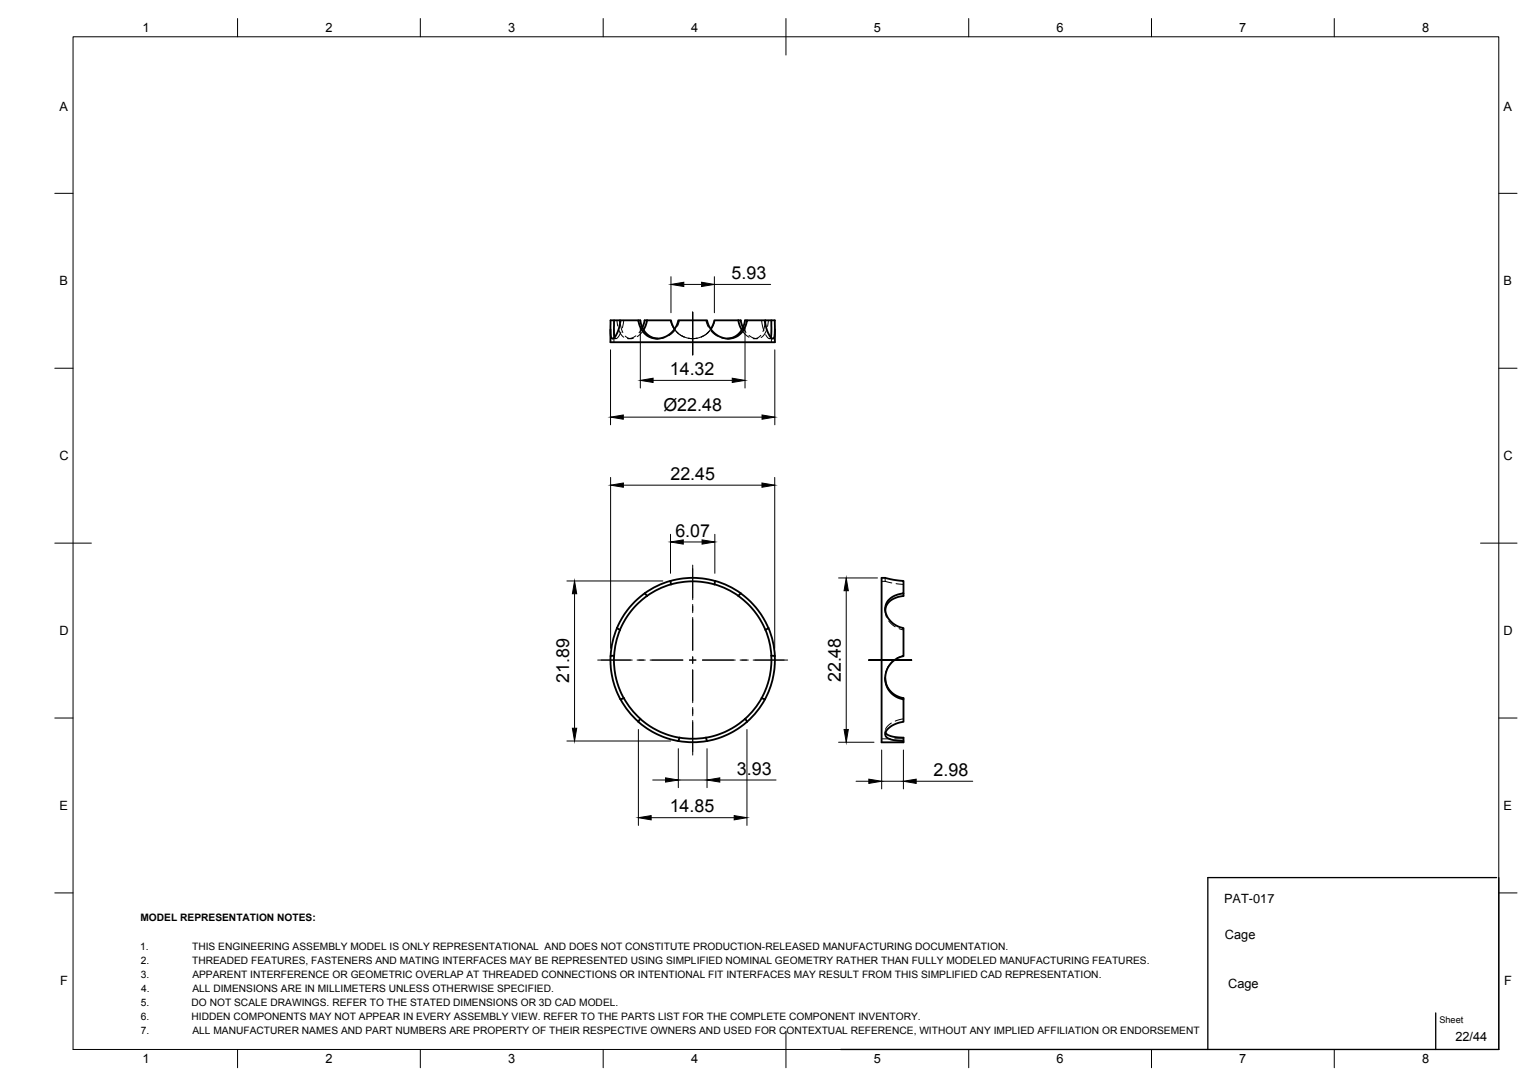
ISO-10303-21;
HEADER;
/* Generated by software containing ST-Developer
 * from STEP Tools, Inc. (www.steptools.com) 
 */

FILE_DESCRIPTION(
/* description */ ('Cam-and-follower valve demonstrator'),
/* implementation_level */ '2;1');

FILE_NAME(
/* name */ 'Cage.step',
/* time_stamp */ '2026-10-28T03:25:17-07:00',
/* author */ (''),
/* organization */ (''),
/* preprocessor_version */ 'ST-DEVELOPER v20.2',
/* originating_system */ 'Autodesk Translation Framework v15.17.0.0',
/* authorisation */ '');

FILE_SCHEMA (('AUTOMOTIVE_DESIGN { 1 0 10303 214 3 1 1 }'));
ENDSEC;

DATA;
#10=MECHANICAL_DESIGN_GEOMETRIC_PRESENTATION_REPRESENTATION('',(#433),#12896);
#300=SPHERICAL_SURFACE('',#6971,0.309556);
#301=SPHERICAL_SURFACE('',#6987,0.309556);
#302=SPHERICAL_SURFACE('',#6992,0.309556);
#303=SPHERICAL_SURFACE('',#6998,0.309556);
#304=SPHERICAL_SURFACE('',#7003,0.309556);
#305=SPHERICAL_SURFACE('',#7008,0.309556);
#306=SPHERICAL_SURFACE('',#7016,0.309556);
#325=B_SPLINE_CURVE_WITH_KNOTS('',3,(#11597,#11598,#11599,#11600,#11601,
#11602,#11603,#11604,#11605,#11606,#11607,#11608,#11609,#11610,#11611,#11612,
#11613,#11614,#11615,#11616,#11617,#11618),.UNSPECIFIED.,.F.,.F.,(4,2,2,
2,2,2,2,2,2,2,4),(0.0591825211272536,0.157966726598481,0.236950089897721,
0.315933453196962,0.391576304923761,0.46721915665056,0.54286200837736,0.618504860104159,
0.697488223403399,0.77647158670264,0.875255792173867),.UNSPECIFIED.);
#326=B_SPLINE_CURVE_WITH_KNOTS('',3,(#11622,#11623,#11624,#11625,#11626,
#11627,#11628,#11629,#11630,#11631,#11632,#11633,#11634,#11635,#11636,#11637,
#11638,#11639,#11640,#11641,#11642,#11643),.UNSPECIFIED.,.F.,.F.,(4,2,2,
2,2,2,2,2,2,2,4),(0.0581119756758434,0.106553146291161,0.213106292582322,
0.30849933801665,0.386091982889075,0.4636846277615,0.541277272633925,0.61886991750635,
0.714262962940678,0.820816109231839,0.869257279847157),.UNSPECIFIED.);
#327=B_SPLINE_CURVE_WITH_KNOTS('',3,(#11649,#11650,#11651,#11652,#11653,
#11654,#11655,#11656,#11657,#11658,#11659,#11660,#11661,#11662,#11663,#11664,
#11665,#11666,#11667,#11668,#11669,#11670),.UNSPECIFIED.,.F.,.F.,(4,2,2,
2,2,2,2,2,2,2,4),(0.0581119756758434,0.106553146291161,0.213106292582322,
0.30849933801665,0.386091982889075,0.4636846277615,0.541277272633925,0.61886991750635,
0.714262962940679,0.820816109231839,0.869257279847157),.UNSPECIFIED.);
#328=B_SPLINE_CURVE_WITH_KNOTS('',3,(#11674,#11675,#11676,#11677,#11678,
#11679,#11680,#11681,#11682,#11683,#11684,#11685,#11686,#11687,#11688,#11689,
#11690,#11691,#11692,#11693,#11694,#11695),.UNSPECIFIED.,.F.,.F.,(4,2,2,
2,2,2,2,2,2,2,4),(0.0581119756758433,0.106553146291161,0.213106292582322,
0.308499338016649,0.386091982889075,0.4636846277615,0.541277272633925,0.61886991750635,
0.714262962940678,0.820816109231839,0.869257279847157),.UNSPECIFIED.);
#329=B_SPLINE_CURVE_WITH_KNOTS('',3,(#11704,#11705,#11706,#11707,#11708,
#11709,#11710,#11711,#11712,#11713,#11714,#11715,#11716,#11717,#11718,#11719,
#11720,#11721,#11722,#11723,#11724,#11725),.UNSPECIFIED.,.F.,.F.,(4,2,2,
2,2,2,2,2,2,2,4),(0.0581119756758433,0.106553146291161,0.213106292582322,
0.30849933801665,0.386091982889075,0.4636846277615,0.541277272633925,0.61886991750635,
0.714262962940678,0.820816109231839,0.869257279847157),.UNSPECIFIED.);
#330=B_SPLINE_CURVE_WITH_KNOTS('',3,(#11729,#11730,#11731,#11732,#11733,
#11734,#11735,#11736,#11737,#11738,#11739,#11740,#11741,#11742,#11743,#11744,
#11745,#11746,#11747,#11748,#11749,#11750),.UNSPECIFIED.,.F.,.F.,(4,2,2,
2,2,2,2,2,2,2,4),(0.0581119756758434,0.106553146291161,0.213106292582322,
0.30849933801665,0.386091982889075,0.4636846277615,0.541277272633925,0.61886991750635,
0.714262962940678,0.820816109231839,0.869257279847157),.UNSPECIFIED.);
#331=B_SPLINE_CURVE_WITH_KNOTS('',3,(#11754,#11755,#11756,#11757,#11758,
#11759,#11760,#11761,#11762,#11763,#11764,#11765,#11766,#11767,#11768,#11769,
#11770,#11771,#11772,#11773,#11774,#11775),.UNSPECIFIED.,.F.,.F.,(4,2,2,
2,2,2,2,2,2,2,4),(0.0581119756758434,0.106553146291161,0.213106292582322,
0.30849933801665,0.386091982889075,0.4636846277615,0.541277272633925,0.61886991750635,
0.714262962940678,0.820816109231839,0.869257279847157),.UNSPECIFIED.);
#332=B_SPLINE_CURVE_WITH_KNOTS('',3,(#11779,#11780,#11781,#11782,#11783,
#11784,#11785,#11786,#11787,#11788,#11789,#11790,#11791,#11792,#11793,#11794,
#11795,#11796,#11797,#11798,#11799,#11800),.UNSPECIFIED.,.F.,.F.,(4,2,2,
2,2,2,2,2,2,2,4),(0.0581119756758433,0.106553146291161,0.213106292582322,
0.30849933801665,0.386091982889075,0.4636846277615,0.541277272633925,0.61886991750635,
0.714262962940678,0.820816109231839,0.869257279847157),.UNSPECIFIED.);
#333=B_SPLINE_CURVE_WITH_KNOTS('',3,(#11808,#11809,#11810,#11811,#11812,
#11813,#11814,#11815,#11816,#11817,#11818,#11819,#11820,#11821,#11822,#11823,
#11824,#11825,#11826,#11827,#11828,#11829),.UNSPECIFIED.,.F.,.F.,(4,2,2,
2,2,2,2,2,2,2,4),(0.0591825211272536,0.157966726598481,0.236950089897721,
0.315933453196962,0.391576304923761,0.467219156650561,0.54286200837736,
0.618504860104159,0.697488223403399,0.77647158670264,0.875255792173867),
 .UNSPECIFIED.);
#334=B_SPLINE_CURVE_WITH_KNOTS('',3,(#11837,#11838,#11839,#11840,#11841,
#11842,#11843,#11844,#11845,#11846,#11847,#11848,#11849,#11850,#11851,#11852,
#11853,#11854,#11855,#11856,#11857,#11858),.UNSPECIFIED.,.F.,.F.,(4,2,2,
2,2,2,2,2,2,2,4),(0.0591825211272536,0.157966726598481,0.236950089897722,
0.315933453196962,0.391576304923761,0.467219156650561,0.54286200837736,
0.618504860104159,0.697488223403399,0.77647158670264,0.875255792173867),
 .UNSPECIFIED.);
#335=B_SPLINE_CURVE_WITH_KNOTS('',3,(#11868,#11869,#11870,#11871,#11872,
#11873,#11874,#11875,#11876,#11877,#11878,#11879,#11880,#11881,#11882,#11883,
#11884,#11885,#11886,#11887,#11888,#11889),.UNSPECIFIED.,.F.,.F.,(4,2,2,
2,2,2,2,2,2,2,4),(0.0591825211272536,0.157966726598481,0.236950089897721,
0.315933453196962,0.391576304923761,0.46721915665056,0.54286200837736,0.618504860104159,
0.697488223403399,0.77647158670264,0.875255792173867),.UNSPECIFIED.);
#336=B_SPLINE_CURVE_WITH_KNOTS('',3,(#11897,#11898,#11899,#11900,#11901,
#11902,#11903,#11904,#11905,#11906,#11907,#11908,#11909,#11910,#11911,#11912,
#11913,#11914,#11915,#11916,#11917,#11918),.UNSPECIFIED.,.F.,.F.,(4,2,2,
2,2,2,2,2,2,2,4),(0.0591825211272536,0.157966726598481,0.236950089897721,
0.315933453196962,0.391576304923761,0.46721915665056,0.542862008377359,
0.618504860104159,0.697488223403399,0.776471586702639,0.875255792173867),
 .UNSPECIFIED.);
#337=B_SPLINE_CURVE_WITH_KNOTS('',3,(#11926,#11927,#11928,#11929,#11930,
#11931,#11932,#11933,#11934,#11935,#11936,#11937,#11938,#11939,#11940,#11941,
#11942,#11943,#11944,#11945,#11946,#11947),.UNSPECIFIED.,.F.,.F.,(4,2,2,
2,2,2,2,2,2,2,4),(0.0591825211272536,0.157966726598481,0.236950089897721,
0.315933453196962,0.391576304923761,0.46721915665056,0.54286200837736,0.618504860104159,
0.697488223403399,0.77647158670264,0.875255792173867),.UNSPECIFIED.);
#338=B_SPLINE_CURVE_WITH_KNOTS('',3,(#11956,#11957,#11958,#11959,#11960,
#11961,#11962,#11963,#11964,#11965,#11966,#11967,#11968,#11969,#11970,#11971,
#11972,#11973,#11974,#11975,#11976,#11977),.UNSPECIFIED.,.F.,.F.,(4,2,2,
2,2,2,2,2,2,2,4),(0.0591825211272536,0.157966726598481,0.236950089897721,
0.315933453196962,0.391576304923761,0.46721915665056,0.542862008377359,
0.618504860104159,0.697488223403399,0.776471586702639,0.875255792173867),
 .UNSPECIFIED.);
#355=SHAPE_REPRESENTATION_RELATIONSHIP('SRR','None',#13072,#391);
#391=ADVANCED_BREP_SHAPE_REPRESENTATION('',(#476),#12872);
#433=STYLED_ITEM('',(#13330),#476);
#476=MANIFOLD_SOLID_BREP('Continuous crown cage',#6200);
#608=FACE_BOUND('',#1762,.T.);
#820=CIRCLE('',#6972,0.303778037777585);
#821=CIRCLE('',#6973,0.303778037777585);
#822=CIRCLE('',#6975,1.123812);
#823=CIRCLE('',#6976,1.123812);
#824=CIRCLE('',#6977,1.123812);
#825=CIRCLE('',#6978,1.123812);
#826=CIRCLE('',#6979,1.123812);
#827=CIRCLE('',#6980,1.123812);
#828=CIRCLE('',#6981,1.123812);
#829=CIRCLE('',#6982,1.123812);
#830=CIRCLE('',#6983,1.123812);
#831=CIRCLE('',#6985,1.076188);
#832=CIRCLE('',#6986,0.303778037777585);
#833=CIRCLE('',#6988,0.303778037777585);
#834=CIRCLE('',#6990,1.076188);
#835=CIRCLE('',#6991,0.303778037777585);
#836=CIRCLE('',#6993,0.303778037777585);
#837=CIRCLE('',#6995,1.076188);
#838=CIRCLE('',#6996,1.076188);
#839=CIRCLE('',#6997,0.303778037777585);
#840=CIRCLE('',#6999,0.303778037777585);
#841=CIRCLE('',#7001,1.076188);
#842=CIRCLE('',#7002,0.303778037777585);
#843=CIRCLE('',#7004,0.303778037777585);
#844=CIRCLE('',#7006,1.076188);
#845=CIRCLE('',#7007,0.303778037777585);
#846=CIRCLE('',#7009,0.303778037777585);
#847=CIRCLE('',#7011,1.076188);
#848=CIRCLE('',#7012,1.076188);
#849=CIRCLE('',#7013,1.076188);
#850=CIRCLE('',#7015,0.303778037777585);
#851=CIRCLE('',#7017,0.303778037777585);
#1044=CYLINDRICAL_SURFACE('',#6974,1.123812);
#1045=CYLINDRICAL_SURFACE('',#7010,1.076188);
#1265=FACE_OUTER_BOUND('',#1746,.T.);
#1266=FACE_OUTER_BOUND('',#1747,.T.);
#1267=FACE_OUTER_BOUND('',#1748,.T.);
#1268=FACE_OUTER_BOUND('',#1749,.T.);
#1269=FACE_OUTER_BOUND('',#1750,.T.);
#1270=FACE_OUTER_BOUND('',#1751,.T.);
#1271=FACE_OUTER_BOUND('',#1752,.T.);
#1272=FACE_OUTER_BOUND('',#1753,.T.);
#1273=FACE_OUTER_BOUND('',#1754,.T.);
#1274=FACE_OUTER_BOUND('',#1755,.T.);
#1275=FACE_OUTER_BOUND('',#1756,.T.);
#1276=FACE_OUTER_BOUND('',#1757,.T.);
#1277=FACE_OUTER_BOUND('',#1758,.T.);
#1278=FACE_OUTER_BOUND('',#1759,.T.);
#1279=FACE_OUTER_BOUND('',#1760,.T.);
#1280=FACE_OUTER_BOUND('',#1761,.T.);
#1281=FACE_OUTER_BOUND('',#1763,.T.);
#1746=EDGE_LOOP('',(#4833,#4834,#4835,#4836));
#1747=EDGE_LOOP('',(#4837,#4838,#4839,#4840,#4841,#4842,#4843,#4844,#4845,
#4846,#4847,#4848,#4849,#4850,#4851,#4852,#4853,#4854));
#1748=EDGE_LOOP('',(#4855,#4856,#4857,#4858));
#1749=EDGE_LOOP('',(#4859,#4860,#4861,#4862));
#1750=EDGE_LOOP('',(#4863,#4864,#4865,#4866));
#1751=EDGE_LOOP('',(#4867,#4868,#4869,#4870));
#1752=EDGE_LOOP('',(#4871,#4872,#4873,#4874,#4875,#4876));
#1753=EDGE_LOOP('',(#4877,#4878,#4879,#4880));
#1754=EDGE_LOOP('',(#4881,#4882,#4883,#4884));
#1755=EDGE_LOOP('',(#4885,#4886,#4887,#4888));
#1756=EDGE_LOOP('',(#4889,#4890,#4891,#4892));
#1757=EDGE_LOOP('',(#4893,#4894,#4895,#4896));
#1758=EDGE_LOOP('',(#4897,#4898,#4899,#4900,#4901,#4902,#4903,#4904,#4905,
#4906,#4907,#4908,#4909,#4910,#4911,#4912,#4913,#4914));
#1759=EDGE_LOOP('',(#4915,#4916,#4917,#4918));
#1760=EDGE_LOOP('',(#4919,#4920,#4921,#4922));
#1761=EDGE_LOOP('',(#4923));
#1762=EDGE_LOOP('',(#4924));
#1763=EDGE_LOOP('',(#4925,#4926,#4927,#4928));
#2202=LINE('',#11699,#2624);
#2203=LINE('',#11952,#2625);
#2624=VECTOR('',#8333,1.123812);
#2625=VECTOR('',#8402,1.076188);
#3093=VERTEX_POINT('',#11595);
#3094=VERTEX_POINT('',#11596);
#3095=VERTEX_POINT('',#11619);
#3096=VERTEX_POINT('',#11621);
#3097=VERTEX_POINT('',#11646);
#3098=VERTEX_POINT('',#11648);
#3099=VERTEX_POINT('',#11671);
#3100=VERTEX_POINT('',#11673);
#3101=VERTEX_POINT('',#11696);
#3102=VERTEX_POINT('',#11698);
#3103=VERTEX_POINT('',#11701);
#3104=VERTEX_POINT('',#11703);
#3105=VERTEX_POINT('',#11726);
#3106=VERTEX_POINT('',#11728);
#3107=VERTEX_POINT('',#11751);
#3108=VERTEX_POINT('',#11753);
#3109=VERTEX_POINT('',#11776);
#3110=VERTEX_POINT('',#11778);
#3111=VERTEX_POINT('',#11803);
#3112=VERTEX_POINT('',#11807);
#3113=VERTEX_POINT('',#11832);
#3114=VERTEX_POINT('',#11836);
#3115=VERTEX_POINT('',#11861);
#3116=VERTEX_POINT('',#11863);
#3117=VERTEX_POINT('',#11867);
#3118=VERTEX_POINT('',#11892);
#3119=VERTEX_POINT('',#11896);
#3120=VERTEX_POINT('',#11921);
#3121=VERTEX_POINT('',#11925);
#3122=VERTEX_POINT('',#11950);
#3123=VERTEX_POINT('',#11953);
#3124=VERTEX_POINT('',#11955);
#3713=EDGE_CURVE('',#3093,#3094,#325,.T.);
#3714=EDGE_CURVE('',#3095,#3093,#820,.T.);
#3715=EDGE_CURVE('',#3096,#3095,#326,.T.);
#3716=EDGE_CURVE('',#3094,#3096,#821,.T.);
#3717=EDGE_CURVE('',#3097,#3095,#822,.T.);
#3718=EDGE_CURVE('',#3097,#3098,#327,.T.);
#3719=EDGE_CURVE('',#3099,#3098,#823,.T.);
#3720=EDGE_CURVE('',#3099,#3100,#328,.T.);
#3721=EDGE_CURVE('',#3101,#3100,#824,.T.);
#3722=EDGE_CURVE('',#3101,#3102,#2202,.T.);
#3723=EDGE_CURVE('',#3102,#3102,#825,.T.);
#3724=EDGE_CURVE('',#3103,#3101,#826,.T.);
#3725=EDGE_CURVE('',#3103,#3104,#329,.T.);
#3726=EDGE_CURVE('',#3105,#3104,#827,.T.);
#3727=EDGE_CURVE('',#3105,#3106,#330,.T.);
#3728=EDGE_CURVE('',#3107,#3106,#828,.T.);
#3729=EDGE_CURVE('',#3107,#3108,#331,.T.);
#3730=EDGE_CURVE('',#3109,#3108,#829,.T.);
#3731=EDGE_CURVE('',#3109,#3110,#332,.T.);
#3732=EDGE_CURVE('',#3096,#3110,#830,.T.);
#3733=EDGE_CURVE('',#3093,#3111,#831,.T.);
#3734=EDGE_CURVE('',#3111,#3097,#832,.T.);
#3735=EDGE_CURVE('',#3112,#3111,#333,.T.);
#3736=EDGE_CURVE('',#3098,#3112,#833,.T.);
#3737=EDGE_CURVE('',#3112,#3113,#834,.T.);
#3738=EDGE_CURVE('',#3113,#3099,#835,.T.);
#3739=EDGE_CURVE('',#3114,#3113,#334,.T.);
#3740=EDGE_CURVE('',#3100,#3114,#836,.T.);
#3741=EDGE_CURVE('',#3114,#3115,#837,.T.);
#3742=EDGE_CURVE('',#3115,#3116,#838,.T.);
#3743=EDGE_CURVE('',#3116,#3103,#839,.T.);
#3744=EDGE_CURVE('',#3117,#3116,#335,.T.);
#3745=EDGE_CURVE('',#3104,#3117,#840,.T.);
#3746=EDGE_CURVE('',#3117,#3118,#841,.T.);
#3747=EDGE_CURVE('',#3118,#3105,#842,.T.);
#3748=EDGE_CURVE('',#3119,#3118,#336,.T.);
#3749=EDGE_CURVE('',#3106,#3119,#843,.T.);
#3750=EDGE_CURVE('',#3119,#3120,#844,.T.);
#3751=EDGE_CURVE('',#3120,#3107,#845,.T.);
#3752=EDGE_CURVE('',#3121,#3120,#337,.T.);
#3753=EDGE_CURVE('',#3108,#3121,#846,.T.);
#3754=EDGE_CURVE('',#3122,#3122,#847,.T.);
#3755=EDGE_CURVE('',#3122,#3115,#2203,.T.);
#3756=EDGE_CURVE('',#3123,#3094,#848,.T.);
#3757=EDGE_CURVE('',#3123,#3124,#338,.T.);
#3758=EDGE_CURVE('',#3121,#3124,#849,.T.);
#3759=EDGE_CURVE('',#3110,#3123,#850,.T.);
#3760=EDGE_CURVE('',#3124,#3109,#851,.T.);
#4833=ORIENTED_EDGE('',*,*,#3713,.F.);
#4834=ORIENTED_EDGE('',*,*,#3714,.F.);
#4835=ORIENTED_EDGE('',*,*,#3715,.F.);
#4836=ORIENTED_EDGE('',*,*,#3716,.F.);
#4837=ORIENTED_EDGE('',*,*,#3715,.T.);
#4838=ORIENTED_EDGE('',*,*,#3717,.F.);
#4839=ORIENTED_EDGE('',*,*,#3718,.T.);
#4840=ORIENTED_EDGE('',*,*,#3719,.F.);
#4841=ORIENTED_EDGE('',*,*,#3720,.T.);
#4842=ORIENTED_EDGE('',*,*,#3721,.F.);
#4843=ORIENTED_EDGE('',*,*,#3722,.T.);
#4844=ORIENTED_EDGE('',*,*,#3723,.F.);
#4845=ORIENTED_EDGE('',*,*,#3722,.F.);
#4846=ORIENTED_EDGE('',*,*,#3724,.F.);
#4847=ORIENTED_EDGE('',*,*,#3725,.T.);
#4848=ORIENTED_EDGE('',*,*,#3726,.F.);
#4849=ORIENTED_EDGE('',*,*,#3727,.T.);
#4850=ORIENTED_EDGE('',*,*,#3728,.F.);
#4851=ORIENTED_EDGE('',*,*,#3729,.T.);
#4852=ORIENTED_EDGE('',*,*,#3730,.F.);
#4853=ORIENTED_EDGE('',*,*,#3731,.T.);
#4854=ORIENTED_EDGE('',*,*,#3732,.F.);
#4855=ORIENTED_EDGE('',*,*,#3714,.T.);
#4856=ORIENTED_EDGE('',*,*,#3733,.T.);
#4857=ORIENTED_EDGE('',*,*,#3734,.T.);
#4858=ORIENTED_EDGE('',*,*,#3717,.T.);
#4859=ORIENTED_EDGE('',*,*,#3735,.F.);
#4860=ORIENTED_EDGE('',*,*,#3736,.F.);
#4861=ORIENTED_EDGE('',*,*,#3718,.F.);
#4862=ORIENTED_EDGE('',*,*,#3734,.F.);
#4863=ORIENTED_EDGE('',*,*,#3736,.T.);
#4864=ORIENTED_EDGE('',*,*,#3737,.T.);
#4865=ORIENTED_EDGE('',*,*,#3738,.T.);
#4866=ORIENTED_EDGE('',*,*,#3719,.T.);
#4867=ORIENTED_EDGE('',*,*,#3739,.F.);
#4868=ORIENTED_EDGE('',*,*,#3740,.F.);
#4869=ORIENTED_EDGE('',*,*,#3720,.F.);
#4870=ORIENTED_EDGE('',*,*,#3738,.F.);
#4871=ORIENTED_EDGE('',*,*,#3740,.T.);
#4872=ORIENTED_EDGE('',*,*,#3741,.T.);
#4873=ORIENTED_EDGE('',*,*,#3742,.T.);
#4874=ORIENTED_EDGE('',*,*,#3743,.T.);
#4875=ORIENTED_EDGE('',*,*,#3724,.T.);
#4876=ORIENTED_EDGE('',*,*,#3721,.T.);
#4877=ORIENTED_EDGE('',*,*,#3744,.F.);
#4878=ORIENTED_EDGE('',*,*,#3745,.F.);
#4879=ORIENTED_EDGE('',*,*,#3725,.F.);
#4880=ORIENTED_EDGE('',*,*,#3743,.F.);
#4881=ORIENTED_EDGE('',*,*,#3745,.T.);
#4882=ORIENTED_EDGE('',*,*,#3746,.T.);
#4883=ORIENTED_EDGE('',*,*,#3747,.T.);
#4884=ORIENTED_EDGE('',*,*,#3726,.T.);
#4885=ORIENTED_EDGE('',*,*,#3748,.F.);
#4886=ORIENTED_EDGE('',*,*,#3749,.F.);
#4887=ORIENTED_EDGE('',*,*,#3727,.F.);
#4888=ORIENTED_EDGE('',*,*,#3747,.F.);
#4889=ORIENTED_EDGE('',*,*,#3749,.T.);
#4890=ORIENTED_EDGE('',*,*,#3750,.T.);
#4891=ORIENTED_EDGE('',*,*,#3751,.T.);
#4892=ORIENTED_EDGE('',*,*,#3728,.T.);
#4893=ORIENTED_EDGE('',*,*,#3729,.F.);
#4894=ORIENTED_EDGE('',*,*,#3751,.F.);
#4895=ORIENTED_EDGE('',*,*,#3752,.F.);
#4896=ORIENTED_EDGE('',*,*,#3753,.F.);
#4897=ORIENTED_EDGE('',*,*,#3754,.F.);
#4898=ORIENTED_EDGE('',*,*,#3755,.T.);
#4899=ORIENTED_EDGE('',*,*,#3741,.F.);
#4900=ORIENTED_EDGE('',*,*,#3739,.T.);
#4901=ORIENTED_EDGE('',*,*,#3737,.F.);
#4902=ORIENTED_EDGE('',*,*,#3735,.T.);
#4903=ORIENTED_EDGE('',*,*,#3733,.F.);
#4904=ORIENTED_EDGE('',*,*,#3713,.T.);
#4905=ORIENTED_EDGE('',*,*,#3756,.F.);
#4906=ORIENTED_EDGE('',*,*,#3757,.T.);
#4907=ORIENTED_EDGE('',*,*,#3758,.F.);
#4908=ORIENTED_EDGE('',*,*,#3752,.T.);
#4909=ORIENTED_EDGE('',*,*,#3750,.F.);
#4910=ORIENTED_EDGE('',*,*,#3748,.T.);
#4911=ORIENTED_EDGE('',*,*,#3746,.F.);
#4912=ORIENTED_EDGE('',*,*,#3744,.T.);
#4913=ORIENTED_EDGE('',*,*,#3742,.F.);
#4914=ORIENTED_EDGE('',*,*,#3755,.F.);
#4915=ORIENTED_EDGE('',*,*,#3716,.T.);
#4916=ORIENTED_EDGE('',*,*,#3732,.T.);
#4917=ORIENTED_EDGE('',*,*,#3759,.T.);
#4918=ORIENTED_EDGE('',*,*,#3756,.T.);
#4919=ORIENTED_EDGE('',*,*,#3731,.F.);
#4920=ORIENTED_EDGE('',*,*,#3760,.F.);
#4921=ORIENTED_EDGE('',*,*,#3757,.F.);
#4922=ORIENTED_EDGE('',*,*,#3759,.F.);
#4923=ORIENTED_EDGE('',*,*,#3723,.T.);
#4924=ORIENTED_EDGE('',*,*,#3754,.T.);
#4925=ORIENTED_EDGE('',*,*,#3753,.T.);
#4926=ORIENTED_EDGE('',*,*,#3758,.T.);
#4927=ORIENTED_EDGE('',*,*,#3760,.T.);
#4928=ORIENTED_EDGE('',*,*,#3730,.T.);
#5682=PLANE('',#6984);
#5683=PLANE('',#6989);
#5684=PLANE('',#6994);
#5685=PLANE('',#7000);
#5686=PLANE('',#7005);
#5687=PLANE('',#7014);
#5688=PLANE('',#7018);
#5689=PLANE('',#7019);
#5981=ADVANCED_FACE('',(#1265),#300,.F.);
#5982=ADVANCED_FACE('',(#1266),#1044,.T.);
#5983=ADVANCED_FACE('',(#1267),#5682,.T.);
#5984=ADVANCED_FACE('',(#1268),#301,.F.);
#5985=ADVANCED_FACE('',(#1269),#5683,.T.);
#5986=ADVANCED_FACE('',(#1270),#302,.F.);
#5987=ADVANCED_FACE('',(#1271),#5684,.T.);
#5988=ADVANCED_FACE('',(#1272),#303,.F.);
#5989=ADVANCED_FACE('',(#1273),#5685,.T.);
#5990=ADVANCED_FACE('',(#1274),#304,.F.);
#5991=ADVANCED_FACE('',(#1275),#5686,.T.);
#5992=ADVANCED_FACE('',(#1276),#305,.F.);
#5993=ADVANCED_FACE('',(#1277),#1045,.F.);
#5994=ADVANCED_FACE('',(#1278),#5687,.T.);
#5995=ADVANCED_FACE('',(#1279),#306,.F.);
#5996=ADVANCED_FACE('',(#1280,#608),#5688,.T.);
#5997=ADVANCED_FACE('',(#1281),#5689,.T.);
#6200=CLOSED_SHELL('',(#5981,#5982,#5983,#5984,#5985,#5986,#5987,#5988,
#5989,#5990,#5991,#5992,#5993,#5994,#5995,#5996,#5997));
#6970=AXIS2_PLACEMENT_3D('',#11593,#8317,#8318);
#6971=AXIS2_PLACEMENT_3D('',#11594,#8319,#8320);
#6972=AXIS2_PLACEMENT_3D('',#11620,#8321,#8322);
#6973=AXIS2_PLACEMENT_3D('',#11644,#8323,#8324);
#6974=AXIS2_PLACEMENT_3D('',#11645,#8325,#8326);
#6975=AXIS2_PLACEMENT_3D('',#11647,#8327,#8328);
#6976=AXIS2_PLACEMENT_3D('',#11672,#8329,#8330);
#6977=AXIS2_PLACEMENT_3D('',#11697,#8331,#8332);
#6978=AXIS2_PLACEMENT_3D('',#11700,#8334,#8335);
#6979=AXIS2_PLACEMENT_3D('',#11702,#8336,#8337);
#6980=AXIS2_PLACEMENT_3D('',#11727,#8338,#8339);
#6981=AXIS2_PLACEMENT_3D('',#11752,#8340,#8341);
#6982=AXIS2_PLACEMENT_3D('',#11777,#8342,#8343);
#6983=AXIS2_PLACEMENT_3D('',#11801,#8344,#8345);
#6984=AXIS2_PLACEMENT_3D('',#11802,#8346,#8347);
#6985=AXIS2_PLACEMENT_3D('',#11804,#8348,#8349);
#6986=AXIS2_PLACEMENT_3D('',#11805,#8350,#8351);
#6987=AXIS2_PLACEMENT_3D('',#11806,#8352,#8353);
#6988=AXIS2_PLACEMENT_3D('',#11830,#8354,#8355);
#6989=AXIS2_PLACEMENT_3D('',#11831,#8356,#8357);
#6990=AXIS2_PLACEMENT_3D('',#11833,#8358,#8359);
#6991=AXIS2_PLACEMENT_3D('',#11834,#8360,#8361);
#6992=AXIS2_PLACEMENT_3D('',#11835,#8362,#8363);
#6993=AXIS2_PLACEMENT_3D('',#11859,#8364,#8365);
#6994=AXIS2_PLACEMENT_3D('',#11860,#8366,#8367);
#6995=AXIS2_PLACEMENT_3D('',#11862,#8368,#8369);
#6996=AXIS2_PLACEMENT_3D('',#11864,#8370,#8371);
#6997=AXIS2_PLACEMENT_3D('',#11865,#8372,#8373);
#6998=AXIS2_PLACEMENT_3D('',#11866,#8374,#8375);
#6999=AXIS2_PLACEMENT_3D('',#11890,#8376,#8377);
#7000=AXIS2_PLACEMENT_3D('',#11891,#8378,#8379);
#7001=AXIS2_PLACEMENT_3D('',#11893,#8380,#8381);
#7002=AXIS2_PLACEMENT_3D('',#11894,#8382,#8383);
#7003=AXIS2_PLACEMENT_3D('',#11895,#8384,#8385);
#7004=AXIS2_PLACEMENT_3D('',#11919,#8386,#8387);
#7005=AXIS2_PLACEMENT_3D('',#11920,#8388,#8389);
#7006=AXIS2_PLACEMENT_3D('',#11922,#8390,#8391);
#7007=AXIS2_PLACEMENT_3D('',#11923,#8392,#8393);
#7008=AXIS2_PLACEMENT_3D('',#11924,#8394,#8395);
#7009=AXIS2_PLACEMENT_3D('',#11948,#8396,#8397);
#7010=AXIS2_PLACEMENT_3D('',#11949,#8398,#8399);
#7011=AXIS2_PLACEMENT_3D('',#11951,#8400,#8401);
#7012=AXIS2_PLACEMENT_3D('',#11954,#8403,#8404);
#7013=AXIS2_PLACEMENT_3D('',#11978,#8405,#8406);
#7014=AXIS2_PLACEMENT_3D('',#11979,#8407,#8408);
#7015=AXIS2_PLACEMENT_3D('',#11980,#8409,#8410);
#7016=AXIS2_PLACEMENT_3D('',#11981,#8411,#8412);
#7017=AXIS2_PLACEMENT_3D('',#11982,#8413,#8414);
#7018=AXIS2_PLACEMENT_3D('',#11983,#8415,#8416);
#7019=AXIS2_PLACEMENT_3D('',#11984,#8417,#8418);
#8317=DIRECTION('axis',(0.,0.,1.));
#8318=DIRECTION('refdir',(1.,0.,0.));
#8319=DIRECTION('center_axis',(0.,0.,1.));
#8320=DIRECTION('ref_axis',(1.,0.,0.));
#8321=DIRECTION('center_axis',(0.,-1.,0.));
#8322=DIRECTION('ref_axis',(0.,0.,-1.));
#8323=DIRECTION('center_axis',(0.,-1.,0.));
#8324=DIRECTION('ref_axis',(0.,0.,-1.));
#8325=DIRECTION('center_axis',(0.,1.,0.));
#8326=DIRECTION('ref_axis',(1.,0.,0.));
#8327=DIRECTION('center_axis',(0.,1.,0.));
#8328=DIRECTION('ref_axis',(1.,0.,0.));
#8329=DIRECTION('center_axis',(0.,1.,0.));
#8330=DIRECTION('ref_axis',(1.,0.,0.));
#8331=DIRECTION('center_axis',(0.,1.,0.));
#8332=DIRECTION('ref_axis',(1.,0.,0.));
#8333=DIRECTION('',(0.,-1.,0.));
#8334=DIRECTION('center_axis',(0.,-1.,0.));
#8335=DIRECTION('ref_axis',(1.,0.,0.));
#8336=DIRECTION('center_axis',(0.,1.,0.));
#8337=DIRECTION('ref_axis',(1.,0.,0.));
#8338=DIRECTION('center_axis',(0.,1.,0.));
#8339=DIRECTION('ref_axis',(1.,0.,0.));
#8340=DIRECTION('center_axis',(0.,1.,0.));
#8341=DIRECTION('ref_axis',(1.,0.,0.));
#8342=DIRECTION('center_axis',(0.,1.,0.));
#8343=DIRECTION('ref_axis',(1.,0.,0.));
#8344=DIRECTION('center_axis',(0.,1.,0.));
#8345=DIRECTION('ref_axis',(1.,0.,0.));
#8346=DIRECTION('center_axis',(0.,1.,0.));
#8347=DIRECTION('ref_axis',(1.,0.,0.));
#8348=DIRECTION('center_axis',(0.,-1.,0.));
#8349=DIRECTION('ref_axis',(1.,0.,0.));
#8350=DIRECTION('center_axis',(0.,-1.,0.));
#8351=DIRECTION('ref_axis',(0.,0.,-1.));
#8352=DIRECTION('center_axis',(8.96625347776458E-17,0.,1.));
#8353=DIRECTION('ref_axis',(1.,0.,0.));
#8354=DIRECTION('center_axis',(0.,-1.,0.));
#8355=DIRECTION('ref_axis',(0.,0.,-1.));
#8356=DIRECTION('center_axis',(0.,1.,0.));
#8357=DIRECTION('ref_axis',(1.,0.,0.));
#8358=DIRECTION('center_axis',(0.,-1.,0.));
#8359=DIRECTION('ref_axis',(1.,0.,0.));
#8360=DIRECTION('center_axis',(0.,-1.,0.));
#8361=DIRECTION('ref_axis',(0.,0.,-1.));
#8362=DIRECTION('center_axis',(0.,0.,1.));
#8363=DIRECTION('ref_axis',(1.,0.,0.));
#8364=DIRECTION('center_axis',(0.,-1.,0.));
#8365=DIRECTION('ref_axis',(0.,0.,-1.));
#8366=DIRECTION('center_axis',(0.,1.,0.));
#8367=DIRECTION('ref_axis',(1.,0.,0.));
#8368=DIRECTION('center_axis',(0.,-1.,0.));
#8369=DIRECTION('ref_axis',(1.,0.,0.));
#8370=DIRECTION('center_axis',(0.,-1.,0.));
#8371=DIRECTION('ref_axis',(1.,0.,0.));
#8372=DIRECTION('center_axis',(0.,-1.,0.));
#8373=DIRECTION('ref_axis',(0.,0.,-1.));
#8374=DIRECTION('center_axis',(0.,0.,1.));
#8375=DIRECTION('ref_axis',(1.,0.,0.));
#8376=DIRECTION('center_axis',(0.,-1.,0.));
#8377=DIRECTION('ref_axis',(0.,0.,-1.));
#8378=DIRECTION('center_axis',(0.,1.,0.));
#8379=DIRECTION('ref_axis',(1.,0.,0.));
#8380=DIRECTION('center_axis',(0.,-1.,0.));
#8381=DIRECTION('ref_axis',(1.,0.,0.));
#8382=DIRECTION('center_axis',(0.,-1.,0.));
#8383=DIRECTION('ref_axis',(0.,0.,-1.));
#8384=DIRECTION('center_axis',(8.96625347776458E-17,0.,1.));
#8385=DIRECTION('ref_axis',(1.,0.,0.));
#8386=DIRECTION('center_axis',(0.,-1.,0.));
#8387=DIRECTION('ref_axis',(0.,0.,-1.));
#8388=DIRECTION('center_axis',(0.,1.,0.));
#8389=DIRECTION('ref_axis',(1.,0.,0.));
#8390=DIRECTION('center_axis',(0.,-1.,0.));
#8391=DIRECTION('ref_axis',(1.,0.,0.));
#8392=DIRECTION('center_axis',(0.,-1.,0.));
#8393=DIRECTION('ref_axis',(0.,0.,-1.));
#8394=DIRECTION('center_axis',(0.,0.,1.));
#8395=DIRECTION('ref_axis',(1.,0.,0.));
#8396=DIRECTION('center_axis',(0.,-1.,0.));
#8397=DIRECTION('ref_axis',(0.,0.,-1.));
#8398=DIRECTION('center_axis',(0.,1.,0.));
#8399=DIRECTION('ref_axis',(1.,0.,0.));
#8400=DIRECTION('center_axis',(0.,1.,0.));
#8401=DIRECTION('ref_axis',(1.,0.,0.));
#8402=DIRECTION('',(0.,1.,0.));
#8403=DIRECTION('center_axis',(0.,-1.,0.));
#8404=DIRECTION('ref_axis',(1.,0.,0.));
#8405=DIRECTION('center_axis',(0.,-1.,0.));
#8406=DIRECTION('ref_axis',(1.,0.,0.));
#8407=DIRECTION('center_axis',(0.,1.,0.));
#8408=DIRECTION('ref_axis',(1.,0.,0.));
#8409=DIRECTION('center_axis',(0.,-1.,0.));
#8410=DIRECTION('ref_axis',(0.,0.,-1.));
#8411=DIRECTION('center_axis',(0.,0.,1.));
#8412=DIRECTION('ref_axis',(1.,0.,0.));
#8413=DIRECTION('center_axis',(0.,-1.,0.));
#8414=DIRECTION('ref_axis',(0.,0.,-1.));
#8415=DIRECTION('center_axis',(0.,-1.,0.));
#8416=DIRECTION('ref_axis',(-1.,0.,0.));
#8417=DIRECTION('center_axis',(0.,1.,0.));
#8418=DIRECTION('ref_axis',(1.,0.,0.));
#11593=CARTESIAN_POINT('',(0.,0.,0.));
#11594=CARTESIAN_POINT('Origin',(0.685838782044607,0.,0.860014630714833));
#11595=CARTESIAN_POINT('',(0.413083465285518,-0.05953,0.993751811093549));
#11596=CARTESIAN_POINT('',(0.876916659919095,-0.05953,0.623857181492959));
#11597=CARTESIAN_POINT('Ctrl Pts',(0.413083465285518,-0.05953,0.993751811093549));
#11598=CARTESIAN_POINT('Ctrl Pts',(0.419070565453383,-0.0925528133349865,
0.991263089003441));
#11599=CARTESIAN_POINT('Ctrl Pts',(0.430199341854858,-0.124911173756694,
0.986608710139579));
#11600=CARTESIAN_POINT('Ctrl Pts',(0.457978755888596,-0.177924977804098,
0.973971221090534));
#11601=CARTESIAN_POINT('Ctrl Pts',(0.473077587363685,-0.199697230012983,
0.966820759530997));
#11602=CARTESIAN_POINT('Ctrl Pts',(0.507057380724533,-0.237895043532788,
0.949440676105255));
#11603=CARTESIAN_POINT('Ctrl Pts',(0.525933334162555,-0.254319232363049,
0.939198248544428));
#11604=CARTESIAN_POINT('Ctrl Pts',(0.564362943424238,-0.28018331644634,
0.916597376014514));
#11605=CARTESIAN_POINT('Ctrl Pts',(0.585840553788742,-0.29104845371857,
0.903141581680914));
#11606=CARTESIAN_POINT('Ctrl Pts',(0.629305439856167,-0.30527573347708,
0.873412008702649));
#11607=CARTESIAN_POINT('Ctrl Pts',(0.651278921914856,-0.308638795020976,
0.857118508332695));
#11608=CARTESIAN_POINT('Ctrl Pts',(0.690705563850638,-0.308638795020976,
0.825676810575914));
#11609=CARTESIAN_POINT('Ctrl Pts',(0.711480111898423,-0.30527573347708,
0.807879894508811));
#11610=CARTESIAN_POINT('Ctrl Pts',(0.750136149454208,-0.29104845371857,
0.772120216227122));
#11611=CARTESIAN_POINT('Ctrl Pts',(0.768033796848072,-0.28018331644634,
0.754175290318038));
#11612=CARTESIAN_POINT('Ctrl Pts',(0.798619410861634,-0.254319232363049,
0.721738358858166));
#11613=CARTESIAN_POINT('Ctrl Pts',(0.812805334167529,-0.237895043532788,
0.705614819529209));
#11614=CARTESIAN_POINT('Ctrl Pts',(0.837310877969633,-0.199697230012983,
0.676354402927683));
#11615=CARTESIAN_POINT('Ctrl Pts',(0.847641868610495,-0.177924977804098,
0.663225258065736));
#11616=CARTESIAN_POINT('Ctrl Pts',(0.866144010579847,-0.124911173756694,
0.638954437806245));
#11617=CARTESIAN_POINT('Ctrl Pts',(0.873158080166742,-0.0925528133349865,
0.62914037979579));
#11618=CARTESIAN_POINT('Ctrl Pts',(0.876916659919095,-0.05953,0.623857181492959));
#11619=CARTESIAN_POINT('',(0.437601487681057,-0.05953,1.03511272300331));
#11620=CARTESIAN_POINT('Origin',(0.685838782044607,-0.05953,0.860014630714833));
#11621=CARTESIAN_POINT('',(0.911784794170997,-0.05953,0.656964154625313));
#11622=CARTESIAN_POINT('Ctrl Pts',(0.911784794170998,-0.0595300000000001,
0.656964154625312));
#11623=CARTESIAN_POINT('Ctrl Pts',(0.909827729890942,-0.0762225747374255,
0.659680317203144));
#11624=CARTESIAN_POINT('Ctrl Pts',(0.907004864562642,-0.0928409665394228,
0.663576540841106));
#11625=CARTESIAN_POINT('Ctrl Pts',(0.895234408667242,-0.144299303100741,
0.679480524217551));
#11626=CARTESIAN_POINT('Ctrl Pts',(0.882797231409153,-0.177024326825049,
0.695831250979106));
#11627=CARTESIAN_POINT('Ctrl Pts',(0.854332839576145,-0.227269801620064,
0.73042219438957));
#11628=CARTESIAN_POINT('Ctrl Pts',(0.834863020612702,-0.251265615809407,
0.752807465209441));
#11629=CARTESIAN_POINT('Ctrl Pts',(0.800439809856111,-0.279889827963178,
0.789147407129766));
#11630=CARTESIAN_POINT('Ctrl Pts',(0.781998747691871,-0.290879136862659,
0.80756613568454));
#11631=CARTESIAN_POINT('Ctrl Pts',(0.742239891936898,-0.305251990234487,
0.844254137480382));
#11632=CARTESIAN_POINT('Ctrl Pts',(0.720906778729541,-0.308638795020976,
0.862505527716294));
#11633=CARTESIAN_POINT('Ctrl Pts',(0.680463863683392,-0.308638795020976,
0.894757676234429));
#11634=CARTESIAN_POINT('Ctrl Pts',(0.657923009631182,-0.305251990234488,
0.91149460735272));
#11635=CARTESIAN_POINT('Ctrl Pts',(0.613307674922609,-0.290879136862659,
0.942092777160053));
#11636=CARTESIAN_POINT('Ctrl Pts',(0.591247219971725,-0.279889827963178,
0.955972930713954));
#11637=CARTESIAN_POINT('Ctrl Pts',(0.548158511259202,-0.251265615809407,
0.981446681891443));
#11638=CARTESIAN_POINT('Ctrl Pts',(0.522002043615455,-0.227269801620063,
0.995447160474328));
#11639=CARTESIAN_POINT('Ctrl Pts',(0.481944444320713,-0.177024326825049,
1.01550068154148));
#11640=CARTESIAN_POINT('Ctrl Pts',(0.463236132117164,-0.14429930310074,
1.0239876538093));
#11641=CARTESIAN_POINT('Ctrl Pts',(0.445111721969657,-0.0928409665394226,
1.03192403056628));
#11642=CARTESIAN_POINT('Ctrl Pts',(0.440685038163619,-0.0762225747374254,
1.03380912944435));
#11643=CARTESIAN_POINT('Ctrl Pts',(0.437601487681056,-0.05953,1.03511272300331));
#11644=CARTESIAN_POINT('Origin',(0.685838782044607,-0.05953,0.860014630714833));
#11645=CARTESIAN_POINT('Origin',(0.,-0.208355,0.));
#11646=CARTESIAN_POINT('',(0.0548532617164168,-0.05953,1.12247250791415));
#11647=CARTESIAN_POINT('Origin',(0.,-0.05953,0.));
#11648=CARTESIAN_POINT('',(-0.536443649899848,-0.05953,0.987512846410683));
#11649=CARTESIAN_POINT('Ctrl Pts',(0.0548532617164173,-0.0595300000000001,
1.12247250791414));
#11650=CARTESIAN_POINT('Ctrl Pts',(0.05150947068137,-0.0762225747374254,
1.12263591311425));
#11651=CARTESIAN_POINT('Ctrl Pts',(0.0467032526342597,-0.0928409665394227,
1.12285816383385));
#11652=CARTESIAN_POINT('Ctrl Pts',(0.0269302585198975,-0.144299303100741,
1.12357162229597));
#11653=CARTESIAN_POINT('Ctrl Pts',(0.006392292392153,-0.177024326825049,
1.12404235695137));
#11654=CARTESIAN_POINT('Ctrl Pts',(-0.0383992541984087,-0.227269801620063,
1.12335509974011));
#11655=CARTESIAN_POINT('Ctrl Pts',(-0.0680399972366993,-0.251265615809407,
1.12208997038458));
#11656=CARTESIAN_POINT('Ctrl Pts',(-0.117914228755037,-0.279889827963178,
1.1178344036749));
#11657=CARTESIAN_POINT('Ctrl Pts',(-0.14381238480104,-0.290879136862659,
1.11490049012186));
#11658=CARTESIAN_POINT('Ctrl Pts',(-0.19728546073067,-0.305251990234488,
1.10669035995599));
#11659=CARTESIAN_POINT('Ctrl Pts',(-0.224855950742601,-0.308638795020976,
1.10139101611326));
#11660=CARTESIAN_POINT('Ctrl Pts',(-0.275287440920027,-0.308638795020976,
1.0898803575765));
#11661=CARTESIAN_POINT('Ctrl Pts',(-0.302426893214945,-0.305251990234488,
1.08269251410343));
#11662=CARTESIAN_POINT('Ctrl Pts',(-0.35416671187353,-0.290879136862659,
1.06688848765783));
#11663=CARTESIAN_POINT('Ctrl Pts',(-0.3787731215897,-0.279889827963178,
1.05829506364875));
#11664=CARTESIAN_POINT('Ctrl Pts',(-0.425554672694338,-0.251265615809407,
1.04048957871266));
#11665=CARTESIAN_POINT('Ctrl Pts',(-0.452808978448581,-0.227269801620063,
1.02876878445619));
#11666=CARTESIAN_POINT('Ctrl Pts',(-0.493462957200432,-0.177024326825049,
1.0099536580922));
#11667=CARTESIAN_POINT('Ctrl Pts',(-0.511762781179148,-0.14429930310074,
1.00061845128527));
#11668=CARTESIAN_POINT('Ctrl Pts',(-0.529268075276157,-0.0928409665394226,
0.991396466802468));
#11669=CARTESIAN_POINT('Ctrl Pts',(-0.533501897135713,-0.0762225747374254,
0.989110885965947));
#11670=CARTESIAN_POINT('Ctrl Pts',(-0.536443649899848,-0.0595300000000001,
0.987512846410683));
#11671=CARTESIAN_POINT('',(-0.843383895613249,-0.05953,0.742736168477219));
#11672=CARTESIAN_POINT('Origin',(0.,-0.05953,0.));
#11673=CARTESIAN_POINT('',(-1.10653577764992,-0.05953,0.196295654879792));
#11674=CARTESIAN_POINT('Ctrl Pts',(-0.843383895613249,-0.0595300000000001,
0.742736168477219));
#11675=CARTESIAN_POINT('Ctrl Pts',(-0.84559647055299,-0.0762225747374255,
0.740223768851062));
#11676=CARTESIAN_POINT('Ctrl Pts',(-0.848766861100456,-0.0928409665394227,
0.736604687327351));
#11677=CARTESIAN_POINT('Ctrl Pts',(-0.861652925570091,-0.144299303100741,
0.721590372101268));
#11678=CARTESIAN_POINT('Ctrl Pts',(-0.87482617317514,-0.177024326825049,
0.705826641853758));
#11679=CARTESIAN_POINT('Ctrl Pts',(-0.902215926359523,-0.227269801620063,
0.670378702718353));
#11680=CARTESIAN_POINT('Ctrl Pts',(-0.919707509403859,-0.251265615809407,
0.646415841396062));
#11681=CARTESIAN_POINT('Ctrl Pts',(-0.947476448101718,-0.279889827963178,
0.604769294586516));
#11682=CARTESIAN_POINT('Ctrl Pts',(-0.961329858300736,-0.290879136862659,
0.582692035672022));
#11683=CARTESIAN_POINT('Ctrl Pts',(-0.988250837578047,-0.305251990234488,
0.535766169015486));
#11684=CARTESIAN_POINT('Ctrl Pts',(-1.00129756308006,-0.308638795020976,
0.510906605094603));
#11685=CARTESIAN_POINT('Ctrl Pts',(-1.02374168767024,-0.308638795020976,
0.46430090015576));
#11686=CARTESIAN_POINT('Ctrl Pts',(-1.03504317708586,-0.305251990234488,
0.438600874831839));
#11687=CARTESIAN_POINT('Ctrl Pts',(-1.05494634094458,-0.290879136862659,
0.388295406390235));
#11688=CARTESIAN_POINT('Ctrl Pts',(-1.06356957703048,-0.279889827963178,
0.363699428370917));
#11689=CARTESIAN_POINT('Ctrl Pts',(-1.0788165083757,-0.251265615809407,
0.316022600643821));
#11690=CARTESIAN_POINT('Ctrl Pts',(-1.08664560412098,-0.227269801620063,
0.287406530683752));
#11691=CARTESIAN_POINT('Ctrl Pts',(-1.09728268713976,-0.177024326825049,
0.243890930799337));
#11692=CARTESIAN_POINT('Ctrl Pts',(-1.10139388218929,-0.144299303100741,
0.22376314604679));
#11693=CARTESIAN_POINT('Ctrl Pts',(-1.10509821673782,-0.0928409665394227,
0.204327142733961));
#11694=CARTESIAN_POINT('Ctrl Pts',(-1.10595102243643,-0.0762225747374254,
0.199591971170104));
#11695=CARTESIAN_POINT('Ctrl Pts',(-1.10653577764992,-0.0595300000000001,
0.196295654879792));
#11696=CARTESIAN_POINT('',(-1.123812,-0.05953,1.37627276864339E-16));
#11697=CARTESIAN_POINT('Origin',(0.,-0.05953,0.));
#11698=CARTESIAN_POINT('',(-1.123812,-0.35718,1.37627276864339E-16));
#11699=CARTESIAN_POINT('',(-1.123812,-0.208355,1.37627276864339E-16));
#11700=CARTESIAN_POINT('Origin',(0.,-0.35718,0.));
#11701=CARTESIAN_POINT('',(-1.10653577764992,-0.05953,-0.196295654879793));
#11702=CARTESIAN_POINT('Origin',(0.,-0.05953,0.));
#11703=CARTESIAN_POINT('',(-0.843383895613249,-0.05953,-0.742736168477219));
#11704=CARTESIAN_POINT('Ctrl Pts',(-1.10653577764992,-0.0595300000000001,
-0.196295654879792));
#11705=CARTESIAN_POINT('Ctrl Pts',(-1.10595102243643,-0.0762225747374255,
-0.199591971170104));
#11706=CARTESIAN_POINT('Ctrl Pts',(-1.10509821673782,-0.0928409665394228,
-0.204327142733962));
#11707=CARTESIAN_POINT('Ctrl Pts',(-1.10139388218929,-0.144299303100741,
-0.22376314604679));
#11708=CARTESIAN_POINT('Ctrl Pts',(-1.09728268713976,-0.177024326825049,
-0.243890930799338));
#11709=CARTESIAN_POINT('Ctrl Pts',(-1.08664560412098,-0.227269801620063,
-0.287406530683753));
#11710=CARTESIAN_POINT('Ctrl Pts',(-1.0788165083757,-0.251265615809407,
-0.316022600643821));
#11711=CARTESIAN_POINT('Ctrl Pts',(-1.06356957703048,-0.279889827963178,
-0.363699428370918));
#11712=CARTESIAN_POINT('Ctrl Pts',(-1.05494634094458,-0.290879136862659,
-0.388295406390235));
#11713=CARTESIAN_POINT('Ctrl Pts',(-1.03504317708586,-0.305251990234488,
-0.438600874831839));
#11714=CARTESIAN_POINT('Ctrl Pts',(-1.02374168767024,-0.308638795020976,
-0.46430090015576));
#11715=CARTESIAN_POINT('Ctrl Pts',(-1.00129756308006,-0.308638795020976,
-0.510906605094603));
#11716=CARTESIAN_POINT('Ctrl Pts',(-0.988250837578047,-0.305251990234488,
-0.535766169015486));
#11717=CARTESIAN_POINT('Ctrl Pts',(-0.961329858300736,-0.290879136862659,
-0.582692035672022));
#11718=CARTESIAN_POINT('Ctrl Pts',(-0.947476448101718,-0.279889827963178,
-0.604769294586516));
#11719=CARTESIAN_POINT('Ctrl Pts',(-0.919707509403859,-0.251265615809407,
-0.646415841396062));
#11720=CARTESIAN_POINT('Ctrl Pts',(-0.902215926359523,-0.227269801620064,
-0.670378702718353));
#11721=CARTESIAN_POINT('Ctrl Pts',(-0.87482617317514,-0.177024326825049,
-0.705826641853758));
#11722=CARTESIAN_POINT('Ctrl Pts',(-0.861652925570091,-0.144299303100741,
-0.721590372101268));
#11723=CARTESIAN_POINT('Ctrl Pts',(-0.848766861100456,-0.0928409665394229,
-0.736604687327351));
#11724=CARTESIAN_POINT('Ctrl Pts',(-0.84559647055299,-0.0762225747374255,
-0.740223768851063));
#11725=CARTESIAN_POINT('Ctrl Pts',(-0.843383895613249,-0.0595300000000001,
-0.742736168477219));
#11726=CARTESIAN_POINT('',(-0.536443649899847,-0.05953,-0.987512846410683));
#11727=CARTESIAN_POINT('Origin',(0.,-0.05953,0.));
#11728=CARTESIAN_POINT('',(0.0548532617164172,-0.05953,-1.12247250791415));
#11729=CARTESIAN_POINT('Ctrl Pts',(-0.536443649899848,-0.0595300000000001,
-0.987512846410683));
#11730=CARTESIAN_POINT('Ctrl Pts',(-0.533501897135712,-0.0762225747374254,
-0.989110885965947));
#11731=CARTESIAN_POINT('Ctrl Pts',(-0.529268075276156,-0.0928409665394227,
-0.991396466802469));
#11732=CARTESIAN_POINT('Ctrl Pts',(-0.511762781179147,-0.144299303100741,
-1.00061845128527));
#11733=CARTESIAN_POINT('Ctrl Pts',(-0.493462957200432,-0.177024326825049,
-1.0099536580922));
#11734=CARTESIAN_POINT('Ctrl Pts',(-0.45280897844858,-0.227269801620063,
-1.02876878445619));
#11735=CARTESIAN_POINT('Ctrl Pts',(-0.425554672694337,-0.251265615809407,
-1.04048957871266));
#11736=CARTESIAN_POINT('Ctrl Pts',(-0.3787731215897,-0.279889827963178,
-1.05829506364875));
#11737=CARTESIAN_POINT('Ctrl Pts',(-0.354166711873529,-0.290879136862659,
-1.06688848765783));
#11738=CARTESIAN_POINT('Ctrl Pts',(-0.302426893214944,-0.305251990234488,
-1.08269251410343));
#11739=CARTESIAN_POINT('Ctrl Pts',(-0.275287440920027,-0.308638795020976,
-1.0898803575765));
#11740=CARTESIAN_POINT('Ctrl Pts',(-0.224855950742601,-0.308638795020976,
-1.10139101611326));
#11741=CARTESIAN_POINT('Ctrl Pts',(-0.19728546073067,-0.305251990234488,
-1.10669035995599));
#11742=CARTESIAN_POINT('Ctrl Pts',(-0.143812384801039,-0.290879136862659,
-1.11490049012186));
#11743=CARTESIAN_POINT('Ctrl Pts',(-0.117914228755037,-0.279889827963178,
-1.1178344036749));
#11744=CARTESIAN_POINT('Ctrl Pts',(-0.0680399972366989,-0.251265615809407,
-1.12208997038458));
#11745=CARTESIAN_POINT('Ctrl Pts',(-0.0383992541984084,-0.227269801620063,
-1.12335509974011));
#11746=CARTESIAN_POINT('Ctrl Pts',(0.00639229239215326,-0.177024326825049,
-1.12404235695137));
#11747=CARTESIAN_POINT('Ctrl Pts',(0.0269302585198977,-0.144299303100741,
-1.12357162229597));
#11748=CARTESIAN_POINT('Ctrl Pts',(0.04670325263426,-0.0928409665394228,
-1.12285816383385));
#11749=CARTESIAN_POINT('Ctrl Pts',(0.0515094706813703,-0.0762225747374255,
-1.12263591311425));
#11750=CARTESIAN_POINT('Ctrl Pts',(0.0548532617164176,-0.0595300000000001,
-1.12247250791414));
#11751=CARTESIAN_POINT('',(0.437601487681057,-0.05953,-1.03511272300331));
#11752=CARTESIAN_POINT('Origin',(0.,-0.05953,0.));
#11753=CARTESIAN_POINT('',(0.911784794170997,-0.05953,-0.656964154625313));
#11754=CARTESIAN_POINT('Ctrl Pts',(0.437601487681056,-0.0595300000000001,
-1.03511272300331));
#11755=CARTESIAN_POINT('Ctrl Pts',(0.440685038163619,-0.0762225747374255,
-1.03380912944435));
#11756=CARTESIAN_POINT('Ctrl Pts',(0.445111721969657,-0.0928409665394228,
-1.03192403056628));
#11757=CARTESIAN_POINT('Ctrl Pts',(0.463236132117164,-0.144299303100741,
-1.0239876538093));
#11758=CARTESIAN_POINT('Ctrl Pts',(0.481944444320713,-0.177024326825049,
-1.01550068154148));
#11759=CARTESIAN_POINT('Ctrl Pts',(0.522002043615455,-0.227269801620064,
-0.995447160474328));
#11760=CARTESIAN_POINT('Ctrl Pts',(0.548158511259203,-0.251265615809407,
-0.981446681891443));
#11761=CARTESIAN_POINT('Ctrl Pts',(0.591247219971725,-0.279889827963178,
-0.955972930713954));
#11762=CARTESIAN_POINT('Ctrl Pts',(0.613307674922609,-0.290879136862659,
-0.942092777160053));
#11763=CARTESIAN_POINT('Ctrl Pts',(0.657923009631182,-0.305251990234487,
-0.91149460735272));
#11764=CARTESIAN_POINT('Ctrl Pts',(0.680463863683393,-0.308638795020976,
-0.894757676234429));
#11765=CARTESIAN_POINT('Ctrl Pts',(0.720906778729542,-0.308638795020976,
-0.862505527716294));
#11766=CARTESIAN_POINT('Ctrl Pts',(0.742239891936899,-0.305251990234488,
-0.844254137480381));
#11767=CARTESIAN_POINT('Ctrl Pts',(0.781998747691872,-0.290879136862659,
-0.80756613568454));
#11768=CARTESIAN_POINT('Ctrl Pts',(0.800439809856112,-0.279889827963178,
-0.789147407129765));
#11769=CARTESIAN_POINT('Ctrl Pts',(0.834863020612702,-0.251265615809407,
-0.752807465209441));
#11770=CARTESIAN_POINT('Ctrl Pts',(0.854332839576145,-0.227269801620064,
-0.73042219438957));
#11771=CARTESIAN_POINT('Ctrl Pts',(0.882797231409153,-0.177024326825049,
-0.695831250979106));
#11772=CARTESIAN_POINT('Ctrl Pts',(0.895234408667242,-0.144299303100741,
-0.679480524217551));
#11773=CARTESIAN_POINT('Ctrl Pts',(0.907004864562642,-0.0928409665394228,
-0.663576540841106));
#11774=CARTESIAN_POINT('Ctrl Pts',(0.909827729890942,-0.0762225747374256,
-0.659680317203144));
#11775=CARTESIAN_POINT('Ctrl Pts',(0.911784794170998,-0.0595300000000001,
-0.656964154625312));
#11776=CARTESIAN_POINT('',(1.08212377959455,-0.05953,-0.303251606722892));
#11777=CARTESIAN_POINT('Origin',(0.,-0.05953,0.));
#11778=CARTESIAN_POINT('',(1.08212377959455,-0.05953,0.303251606722892));
#11779=CARTESIAN_POINT('Ctrl Pts',(1.08212377959455,-0.0595300000000001,
-0.303251606722892));
#11780=CARTESIAN_POINT('Ctrl Pts',(1.0830271513892,-0.0762225747374255,
-0.300028012588062));
#11781=CARTESIAN_POINT('Ctrl Pts',(1.08431331394788,-0.0928409665394228,
-0.2953917518996));
#11782=CARTESIAN_POINT('Ctrl Pts',(1.08940878963422,-0.144299303100741,
-0.276273267473431));
#11783=CARTESIAN_POINT('Ctrl Pts',(1.09443784939331,-0.177024326825049,
-0.256354979351213));
#11784=CARTESIAN_POINT('Ctrl Pts',(1.10373487993589,-0.227269801620064,
-0.212533521233765));
#11785=CARTESIAN_POINT('Ctrl Pts',(1.10909715583869,-0.251265615809407,
-0.183354415742157));
#11786=CARTESIAN_POINT('Ctrl Pts',(1.1160463456491,-0.279889827963178,-0.133783682657561));
#11787=CARTESIAN_POINT('Ctrl Pts',(1.11894887330541,-0.290879136862659,
-0.107881990270302));
#11788=CARTESIAN_POINT('Ctrl Pts',(1.12284346704144,-0.305251990234488,
-0.0539226701638766));
#11789=CARTESIAN_POINT('Ctrl Pts',(1.123812,-0.308638795020976,-0.025864214957475));
#11790=CARTESIAN_POINT('Ctrl Pts',(1.123812,-0.308638795020976,0.025864214957475));
#11791=CARTESIAN_POINT('Ctrl Pts',(1.12284346704144,-0.305251990234488,
0.0539226701638766));
#11792=CARTESIAN_POINT('Ctrl Pts',(1.11894887330541,-0.290879136862659,
0.107881990270302));
#11793=CARTESIAN_POINT('Ctrl Pts',(1.1160463456491,-0.279889827963178,0.133783682657561));
#11794=CARTESIAN_POINT('Ctrl Pts',(1.10909715583869,-0.251265615809407,
0.183354415742157));
#11795=CARTESIAN_POINT('Ctrl Pts',(1.10373487993589,-0.227269801620064,
0.212533521233765));
#11796=CARTESIAN_POINT('Ctrl Pts',(1.09443784939331,-0.177024326825049,
0.256354979351213));
#11797=CARTESIAN_POINT('Ctrl Pts',(1.08940878963422,-0.144299303100741,
0.276273267473431));
#11798=CARTESIAN_POINT('Ctrl Pts',(1.08431331394788,-0.0928409665394228,
0.2953917518996));
#11799=CARTESIAN_POINT('Ctrl Pts',(1.0830271513892,-0.0762225747374255,
0.300028012588062));
#11800=CARTESIAN_POINT('Ctrl Pts',(1.08212377959455,-0.0595300000000001,
0.303251606722892));
#11801=CARTESIAN_POINT('Origin',(0.,-0.05953,0.));
#11802=CARTESIAN_POINT('Origin',(0.,-0.05953,0.));
#11803=CARTESIAN_POINT('',(0.0589974094846122,-0.05953,1.07456964270265));
#11804=CARTESIAN_POINT('Origin',(0.,-0.05953,0.));
#11805=CARTESIAN_POINT('Origin',(-0.244773027351946,-0.05953,1.07242070340001));
#11806=CARTESIAN_POINT('Origin',(-0.244773027351946,0.,1.07242070340001));
#11807=CARTESIAN_POINT('',(-0.519393123750572,-0.05953,0.942555777842682));
#11808=CARTESIAN_POINT('Ctrl Pts',(-0.519393123750572,-0.05953,0.942555777842682));
#11809=CARTESIAN_POINT('Ctrl Pts',(-0.513714466572041,-0.0925528133349865,
0.945684988399766));
#11810=CARTESIAN_POINT('Ctrl Pts',(-0.503136848051455,-0.124911173756694,
0.951483858396181));
#11811=CARTESIAN_POINT('Ctrl Pts',(-0.47593627990192,-0.177924977804098,
0.965323333309091));
#11812=CARTESIAN_POINT('Ctrl Pts',(-0.460931856495794,-0.199697230012983,
0.972669835243841));
#11813=CARTESIAN_POINT('Ctrl Pts',(-0.426157505475872,-0.237895043532788,
0.988400002689705));
#11814=CARTESIAN_POINT('Ctrl Pts',(-0.406380688682952,-0.254319232363049,
0.996771768218699));
#11815=CARTESIAN_POINT('Ctrl Pts',(-0.364750145543744,-0.28018331644634,
1.01272583306292));
#11816=CARTESIAN_POINT('Ctrl Pts',(-0.340838910881557,-0.29104845371857,
1.02112815447116));
#11817=CARTESIAN_POINT('Ctrl Pts',(-0.290495481564827,-0.30527573347708,
1.036574285215));
#11818=CARTESIAN_POINT('Ctrl Pts',(-0.264056468041074,-0.308638795020976,
1.04359501395068));
#11819=CARTESIAN_POINT('Ctrl Pts',(-0.214892249704082,-0.308638795020976,
1.05481642595959));
#11820=CARTESIAN_POINT('Ctrl Pts',(-0.188025341585962,-0.30527573347708,
1.05996242598502));
#11821=CARTESIAN_POINT('Ctrl Pts',(-0.135965654106109,-0.29104845371857,
1.06788913840721));
#11822=CARTESIAN_POINT('Ctrl Pts',(-0.110776745452494,-0.28018331644634,
1.07069360430242));
#11823=CARTESIAN_POINT('Ctrl Pts',(-0.0663467128214646,-0.254319232363049,
1.07438230428002));
#11824=CARTESIAN_POINT('Ctrl Pts',(-0.0448960436540983,-0.237895043532788,
1.07542044338697));
#11825=CARTESIAN_POINT('Ctrl Pts',(-0.00674037211528124,-0.199697230012983,
1.07633607767727));
#11826=CARTESIAN_POINT('Ctrl Pts',(0.00996567398334777,-0.177924977804098,
1.07622728347683));
#11827=CARTESIAN_POINT('Ctrl Pts',(0.0404772621979741,-0.124911173756694,
1.07556023164702));
#11828=CARTESIAN_POINT('Ctrl Pts',(0.0525234025782719,-0.0925528133349865,
1.07492508698591));
#11829=CARTESIAN_POINT('Ctrl Pts',(0.0589974094846124,-0.05953,1.07456964270265));
#11830=CARTESIAN_POINT('Origin',(-0.244773027351946,-0.05953,1.07242070340001));
#11831=CARTESIAN_POINT('Origin',(0.,-0.05953,0.));
#11832=CARTESIAN_POINT('',(-0.803348093619616,-0.05953,0.716109245731214));
#11833=CARTESIAN_POINT('Origin',(0.,-0.05953,0.));
#11834=CARTESIAN_POINT('Origin',(-0.991065754692661,-0.05953,0.477272113029314));
#11835=CARTESIAN_POINT('Origin',(-0.991065754692661,0.,0.477272113029314));
#11836=CARTESIAN_POINT('',(-1.06075609691358,-0.05953,0.181596019242328));
#11837=CARTESIAN_POINT('Ctrl Pts',(-1.06075609691358,-0.05953,0.181596019242328));
#11838=CARTESIAN_POINT('Ctrl Pts',(-1.05966202740332,-0.0925528133349865,
0.187986803072856));
#11839=CARTESIAN_POINT('Ctrl Pts',(-1.05760072925372,-0.124911173756694,
0.199872254546857));
#11840=CARTESIAN_POINT('Ctrl Pts',(-1.05146158959546,-0.177924977804098,
0.22976728653846));
#11841=CARTESIAN_POINT('Ctrl Pts',(-1.04785021111757,-0.199697230012983,
0.246078686169301));
#11842=CARTESIAN_POINT('Ctrl Pts',(-1.03846709802406,-0.237895043532788,
0.283073967563097));
#11843=CARTESIAN_POINT('Ctrl Pts',(-1.03268176429485,-0.254319232363049,
0.303755815985685));
#11844=CARTESIAN_POINT('Ctrl Pts',(-1.01919893537026,-0.28018331644634,
0.346251081972725));
#11845=CARTESIAN_POINT('Ctrl Pts',(-1.01085972381132,-0.29104845371857,
0.370184399726282));
#11846=CARTESIAN_POINT('Ctrl Pts',(-0.99154738033959,-0.30527573347708,
0.419174982698463));
#11847=CARTESIAN_POINT('Ctrl Pts',(-0.980551951791748,-0.308638795020976,
0.444223188605045));
#11848=CARTESIAN_POINT('Ctrl Pts',(-0.958671816228589,-0.308638795020976,
0.489657758261848));
#11849=CARTESIAN_POINT('Ctrl Pts',(-0.945943877838127,-0.30527573347708,
0.51387163140139));
#11850=CARTESIAN_POINT('Ctrl Pts',(-0.91968254693063,-0.29104845371857,
0.559515758398093));
#11851=CARTESIAN_POINT('Ctrl Pts',(-0.906170138993533,-0.28018331644634,
0.580957796077825));
#11852=CARTESIAN_POINT('Ctrl Pts',(-0.8813524085237,-0.254319232363049,
0.617994461173994));
#11853=CARTESIAN_POINT('Ctrl Pts',(-0.868789784891799,-0.237895043532788,
0.635412538795143));
#11854=CARTESIAN_POINT('Ctrl Pts',(-0.845715984518854,-0.199697230012983,
0.66581473268113));
#11855=CARTESIAN_POINT('Ctrl Pts',(-0.835214876415962,-0.177924977804098,
0.678808213394124));
#11856=CARTESIAN_POINT('Ctrl Pts',(-0.815669690204649,-0.124911173756694,
0.702247233627224));
#11857=CARTESIAN_POINT('Ctrl Pts',(-0.807662468433796,-0.0925528133349865,
0.711269279199861));
#11858=CARTESIAN_POINT('Ctrl Pts',(-0.803348093619616,-0.05953,0.716109245731214));
#11859=CARTESIAN_POINT('Origin',(-0.991065754692661,-0.05953,0.477272113029314));
#11860=CARTESIAN_POINT('Origin',(0.,-0.05953,0.));
#11861=CARTESIAN_POINT('',(-1.076188,-0.05953,1.31795018948079E-16));
#11862=CARTESIAN_POINT('Origin',(0.,-0.05953,0.));
#11863=CARTESIAN_POINT('',(-1.06075609691358,-0.05953,-0.181596019242328));
#11864=CARTESIAN_POINT('Origin',(0.,-0.05953,0.));
#11865=CARTESIAN_POINT('Origin',(-0.991065754692661,-0.05953,-0.477272113029314));
#11866=CARTESIAN_POINT('Origin',(-0.991065754692661,0.,-0.477272113029314));
#11867=CARTESIAN_POINT('',(-0.803348093619616,-0.05953,-0.716109245731215));
#11868=CARTESIAN_POINT('Ctrl Pts',(-0.803348093619616,-0.05953,-0.716109245731215));
#11869=CARTESIAN_POINT('Ctrl Pts',(-0.807662468433795,-0.0925528133349865,
-0.711269279199862));
#11870=CARTESIAN_POINT('Ctrl Pts',(-0.815669690204649,-0.124911173756694,
-0.702247233627224));
#11871=CARTESIAN_POINT('Ctrl Pts',(-0.835214876415962,-0.177924977804098,
-0.678808213394124));
#11872=CARTESIAN_POINT('Ctrl Pts',(-0.845715984518854,-0.199697230012983,
-0.66581473268113));
#11873=CARTESIAN_POINT('Ctrl Pts',(-0.868789784891799,-0.237895043532788,
-0.635412538795143));
#11874=CARTESIAN_POINT('Ctrl Pts',(-0.8813524085237,-0.254319232363049,
-0.617994461173994));
#11875=CARTESIAN_POINT('Ctrl Pts',(-0.906170138993533,-0.28018331644634,
-0.580957796077826));
#11876=CARTESIAN_POINT('Ctrl Pts',(-0.91968254693063,-0.29104845371857,
-0.559515758398093));
#11877=CARTESIAN_POINT('Ctrl Pts',(-0.945943877838127,-0.30527573347708,
-0.51387163140139));
#11878=CARTESIAN_POINT('Ctrl Pts',(-0.958671816228589,-0.308638795020976,
-0.489657758261848));
#11879=CARTESIAN_POINT('Ctrl Pts',(-0.980551951791748,-0.308638795020976,
-0.444223188605045));
#11880=CARTESIAN_POINT('Ctrl Pts',(-0.99154738033959,-0.30527573347708,
-0.419174982698463));
#11881=CARTESIAN_POINT('Ctrl Pts',(-1.01085972381132,-0.29104845371857,
-0.370184399726282));
#11882=CARTESIAN_POINT('Ctrl Pts',(-1.01919893537026,-0.28018331644634,
-0.346251081972725));
#11883=CARTESIAN_POINT('Ctrl Pts',(-1.03268176429485,-0.254319232363049,
-0.303755815985685));
#11884=CARTESIAN_POINT('Ctrl Pts',(-1.03846709802406,-0.237895043532788,
-0.283073967563097));
#11885=CARTESIAN_POINT('Ctrl Pts',(-1.04785021111757,-0.199697230012983,
-0.246078686169302));
#11886=CARTESIAN_POINT('Ctrl Pts',(-1.05146158959546,-0.177924977804098,
-0.229767286538461));
#11887=CARTESIAN_POINT('Ctrl Pts',(-1.05760072925372,-0.124911173756694,
-0.199872254546858));
#11888=CARTESIAN_POINT('Ctrl Pts',(-1.05966202740332,-0.0925528133349864,
-0.187986803072857));
#11889=CARTESIAN_POINT('Ctrl Pts',(-1.06075609691358,-0.05953,-0.181596019242328));
#11890=CARTESIAN_POINT('Origin',(-0.991065754692661,-0.05953,-0.477272113029314));
#11891=CARTESIAN_POINT('Origin',(0.,-0.05953,0.));
#11892=CARTESIAN_POINT('',(-0.519393123750572,-0.05953,-0.942555777842682));
#11893=CARTESIAN_POINT('Origin',(0.,-0.05953,0.));
#11894=CARTESIAN_POINT('Origin',(-0.244773027351946,-0.05953,-1.07242070340001));
#11895=CARTESIAN_POINT('Origin',(-0.244773027351946,0.,-1.07242070340001));
#11896=CARTESIAN_POINT('',(0.0589974094846125,-0.05953,-1.07456964270265));
#11897=CARTESIAN_POINT('Ctrl Pts',(0.0589974094846127,-0.05953,-1.07456964270265));
#11898=CARTESIAN_POINT('Ctrl Pts',(0.0525234025782722,-0.0925528133349865,
-1.07492508698591));
#11899=CARTESIAN_POINT('Ctrl Pts',(0.0404772621979744,-0.124911173756694,
-1.07556023164702));
#11900=CARTESIAN_POINT('Ctrl Pts',(0.0099656739833481,-0.177924977804098,
-1.07622728347683));
#11901=CARTESIAN_POINT('Ctrl Pts',(-0.00674037211528096,-0.199697230012983,
-1.07633607767727));
#11902=CARTESIAN_POINT('Ctrl Pts',(-0.044896043654098,-0.237895043532788,
-1.07542044338697));
#11903=CARTESIAN_POINT('Ctrl Pts',(-0.0663467128214644,-0.254319232363049,
-1.07438230428002));
#11904=CARTESIAN_POINT('Ctrl Pts',(-0.110776745452493,-0.28018331644634,
-1.07069360430242));
#11905=CARTESIAN_POINT('Ctrl Pts',(-0.135965654106109,-0.29104845371857,
-1.06788913840721));
#11906=CARTESIAN_POINT('Ctrl Pts',(-0.188025341585962,-0.30527573347708,
-1.05996242598502));
#11907=CARTESIAN_POINT('Ctrl Pts',(-0.214892249704082,-0.308638795020976,
-1.05481642595959));
#11908=CARTESIAN_POINT('Ctrl Pts',(-0.264056468041074,-0.308638795020976,
-1.04359501395068));
#11909=CARTESIAN_POINT('Ctrl Pts',(-0.290495481564827,-0.30527573347708,
-1.036574285215));
#11910=CARTESIAN_POINT('Ctrl Pts',(-0.340838910881557,-0.291048453718569,
-1.02112815447116));
#11911=CARTESIAN_POINT('Ctrl Pts',(-0.364750145543744,-0.28018331644634,
-1.01272583306292));
#11912=CARTESIAN_POINT('Ctrl Pts',(-0.406380688682952,-0.254319232363049,
-0.996771768218699));
#11913=CARTESIAN_POINT('Ctrl Pts',(-0.426157505475872,-0.237895043532788,
-0.988400002689705));
#11914=CARTESIAN_POINT('Ctrl Pts',(-0.460931856495794,-0.199697230012983,
-0.972669835243841));
#11915=CARTESIAN_POINT('Ctrl Pts',(-0.475936279901919,-0.177924977804098,
-0.965323333309091));
#11916=CARTESIAN_POINT('Ctrl Pts',(-0.503136848051454,-0.124911173756694,
-0.951483858396181));
#11917=CARTESIAN_POINT('Ctrl Pts',(-0.513714466572041,-0.0925528133349865,
-0.945684988399766));
#11918=CARTESIAN_POINT('Ctrl Pts',(-0.519393123750572,-0.05953,-0.942555777842682));
#11919=CARTESIAN_POINT('Origin',(-0.244773027351946,-0.05953,-1.07242070340001));
#11920=CARTESIAN_POINT('Origin',(0.,-0.05953,0.));
#11921=CARTESIAN_POINT('',(0.413083465285518,-0.05953,-0.993751811093549));
#11922=CARTESIAN_POINT('Origin',(0.,-0.05953,0.));
#11923=CARTESIAN_POINT('Origin',(0.685838782044607,-0.05953,-0.860014630714833));
#11924=CARTESIAN_POINT('Origin',(0.685838782044607,0.,-0.860014630714833));
#11925=CARTESIAN_POINT('',(0.876916659919095,-0.05953,-0.623857181492959));
#11926=CARTESIAN_POINT('Ctrl Pts',(0.876916659919095,-0.05953,-0.623857181492958));
#11927=CARTESIAN_POINT('Ctrl Pts',(0.873158080166742,-0.0925528133349865,
-0.62914037979579));
#11928=CARTESIAN_POINT('Ctrl Pts',(0.866144010579847,-0.124911173756694,
-0.638954437806245));
#11929=CARTESIAN_POINT('Ctrl Pts',(0.847641868610495,-0.177924977804098,
-0.663225258065736));
#11930=CARTESIAN_POINT('Ctrl Pts',(0.837310877969633,-0.199697230012983,
-0.676354402927683));
#11931=CARTESIAN_POINT('Ctrl Pts',(0.81280533416753,-0.237895043532788,
-0.705614819529209));
#11932=CARTESIAN_POINT('Ctrl Pts',(0.798619410861634,-0.254319232363049,
-0.721738358858166));
#11933=CARTESIAN_POINT('Ctrl Pts',(0.768033796848072,-0.28018331644634,
-0.754175290318038));
#11934=CARTESIAN_POINT('Ctrl Pts',(0.750136149454208,-0.29104845371857,
-0.772120216227122));
#11935=CARTESIAN_POINT('Ctrl Pts',(0.711480111898423,-0.30527573347708,
-0.807879894508811));
#11936=CARTESIAN_POINT('Ctrl Pts',(0.690705563850638,-0.308638795020976,
-0.825676810575913));
#11937=CARTESIAN_POINT('Ctrl Pts',(0.651278921914856,-0.308638795020976,
-0.857118508332695));
#11938=CARTESIAN_POINT('Ctrl Pts',(0.629305439856167,-0.30527573347708,
-0.873412008702649));
#11939=CARTESIAN_POINT('Ctrl Pts',(0.585840553788742,-0.29104845371857,
-0.903141581680914));
#11940=CARTESIAN_POINT('Ctrl Pts',(0.564362943424239,-0.28018331644634,
-0.916597376014514));
#11941=CARTESIAN_POINT('Ctrl Pts',(0.525933334162556,-0.254319232363049,
-0.939198248544427));
#11942=CARTESIAN_POINT('Ctrl Pts',(0.507057380724533,-0.237895043532788,
-0.949440676105255));
#11943=CARTESIAN_POINT('Ctrl Pts',(0.473077587363686,-0.199697230012983,
-0.966820759530997));
#11944=CARTESIAN_POINT('Ctrl Pts',(0.457978755888596,-0.177924977804098,
-0.973971221090534));
#11945=CARTESIAN_POINT('Ctrl Pts',(0.430199341854858,-0.124911173756694,
-0.986608710139579));
#11946=CARTESIAN_POINT('Ctrl Pts',(0.419070565453384,-0.0925528133349865,
-0.991263089003441));
#11947=CARTESIAN_POINT('Ctrl Pts',(0.413083465285518,-0.05953,-0.993751811093549));
#11948=CARTESIAN_POINT('Origin',(0.685838782044607,-0.05953,-0.860014630714833));
#11949=CARTESIAN_POINT('Origin',(0.,-0.208355,0.));
#11950=CARTESIAN_POINT('',(-1.076188,-0.35718,1.31795018948079E-16));
#11951=CARTESIAN_POINT('Origin',(0.,-0.35718,0.));
#11952=CARTESIAN_POINT('',(-1.076188,-0.208355,1.31795018948079E-16));
#11953=CARTESIAN_POINT('',(1.03449977959455,-0.05953,0.296632461748266));
#11954=CARTESIAN_POINT('Origin',(0.,-0.05953,0.));
#11955=CARTESIAN_POINT('',(1.03449977959455,-0.05953,-0.296632461748266));
#11956=CARTESIAN_POINT('Ctrl Pts',(1.03449977959455,-0.05953,0.296632461748267));
#11957=CARTESIAN_POINT('Ctrl Pts',(1.03628691421076,-0.0925528133349865,
0.290399865505497));
#11958=CARTESIAN_POINT('Ctrl Pts',(1.03958665287714,-0.124911173756694,
0.278797079997872));
#11959=CARTESIAN_POINT('Ctrl Pts',(1.0470264474309,-0.177924977804098,0.249198913998601));
#11960=CARTESIAN_POINT('Ctrl Pts',(1.05084995891418,-0.199697230012983,
0.232935932341942));
#11961=CARTESIAN_POINT('Ctrl Pts',(1.05844771715377,-0.237895043532788,
0.195533155353269));
#11962=CARTESIAN_POINT('Ctrl Pts',(1.06220882929878,-0.254319232363049,
0.17438929156337));
#11963=CARTESIAN_POINT('Ctrl Pts',(1.06849922508772,-0.28018331644634,0.130252399648131));
#11964=CARTESIAN_POINT('Ctrl Pts',(1.07137013248666,-0.29104845371857,0.105070977154072));
#11965=CARTESIAN_POINT('Ctrl Pts',(1.07522652957392,-0.30527573347708,0.0525526752791107));
#11966=CARTESIAN_POINT('Ctrl Pts',(1.076188,-0.308638795020976,0.025214283908933));
#11967=CARTESIAN_POINT('Ctrl Pts',(1.076188,-0.308638795020976,-0.025214283908933));
#11968=CARTESIAN_POINT('Ctrl Pts',(1.07522652957392,-0.30527573347708,-0.0525526752791107));
#11969=CARTESIAN_POINT('Ctrl Pts',(1.07137013248666,-0.29104845371857,-0.105070977154072));
#11970=CARTESIAN_POINT('Ctrl Pts',(1.06849922508772,-0.28018331644634,-0.130252399648131));
#11971=CARTESIAN_POINT('Ctrl Pts',(1.06220882929878,-0.254319232363049,
-0.17438929156337));
#11972=CARTESIAN_POINT('Ctrl Pts',(1.05844771715377,-0.237895043532788,
-0.195533155353269));
#11973=CARTESIAN_POINT('Ctrl Pts',(1.05084995891418,-0.199697230012983,
-0.232935932341942));
#11974=CARTESIAN_POINT('Ctrl Pts',(1.0470264474309,-0.177924977804098,-0.249198913998601));
#11975=CARTESIAN_POINT('Ctrl Pts',(1.03958665287714,-0.124911173756694,
-0.278797079997872));
#11976=CARTESIAN_POINT('Ctrl Pts',(1.03628691421076,-0.0925528133349865,
-0.290399865505497));
#11977=CARTESIAN_POINT('Ctrl Pts',(1.03449977959455,-0.05953,-0.296632461748267));
#11978=CARTESIAN_POINT('Origin',(0.,-0.05953,0.));
#11979=CARTESIAN_POINT('Origin',(0.,-0.05953,0.));
#11980=CARTESIAN_POINT('Origin',(1.1,-0.05953,0.));
#11981=CARTESIAN_POINT('Origin',(1.1,0.,0.));
#11982=CARTESIAN_POINT('Origin',(1.1,-0.05953,0.));
#11983=CARTESIAN_POINT('Origin',(0.,-0.35718,0.));
#11984=CARTESIAN_POINT('Origin',(0.,-0.05953,0.));
#12829=UNCERTAINTY_MEASURE_WITH_UNIT(LENGTH_MEASURE(0.001),#12897,
'DISTANCE_ACCURACY_VALUE',
'Maximum model space distance between geometric entities at asserted c
onnectivities');
#12853=UNCERTAINTY_MEASURE_WITH_UNIT(LENGTH_MEASURE(0.001),#12897,
'DISTANCE_ACCURACY_VALUE',
'Maximum model space distance between geometric entities at asserted c
onnectivities');
#12872=(
GEOMETRIC_REPRESENTATION_CONTEXT(3)
GLOBAL_UNCERTAINTY_ASSIGNED_CONTEXT((#12829))
GLOBAL_UNIT_ASSIGNED_CONTEXT((#12897,#12899,#12900))
REPRESENTATION_CONTEXT('','3D')
);
#12896=(
GEOMETRIC_REPRESENTATION_CONTEXT(3)
GLOBAL_UNCERTAINTY_ASSIGNED_CONTEXT((#12853))
GLOBAL_UNIT_ASSIGNED_CONTEXT((#12897,#12899,#12900))
REPRESENTATION_CONTEXT('','3D')
);
#12897=(
LENGTH_UNIT()
NAMED_UNIT(*)
SI_UNIT(.CENTI.,.METRE.)
);
#12899=(
NAMED_UNIT(*)
PLANE_ANGLE_UNIT()
SI_UNIT($,.RADIAN.)
);
#12900=(
NAMED_UNIT(*)
SI_UNIT($,.STERADIAN.)
SOLID_ANGLE_UNIT()
);
#12919=SHAPE_DEFINITION_REPRESENTATION(#12961,#13072);
#12961=PRODUCT_DEFINITION_SHAPE('',$,#13115);
#13072=SHAPE_REPRESENTATION('',(#6970),#12872);
#13096=PRODUCT_DEFINITION_CONTEXT('part definition',#13224,'design');
#13115=PRODUCT_DEFINITION('Cage','Cage',#13157,#13096);
#13157=PRODUCT_DEFINITION_FORMATION('',$,#13244);
#13224=APPLICATION_CONTEXT(
'Core Data for Automotive Mechanical Design Process');
#13225=PRODUCT_CONTEXT('part definition',#13224,'mechanical');
#13244=PRODUCT('Cage','Cage','Cage',(#13225));
#13324=COLOUR_RGB('Grey',0.48,0.52,0.57);
#13325=FILL_AREA_STYLE_COLOUR('',#13324);
#13326=FILL_AREA_STYLE('',(#13325));
#13327=SURFACE_STYLE_FILL_AREA(#13326);
#13328=SURFACE_SIDE_STYLE('',(#13327));
#13329=SURFACE_STYLE_USAGE(.BOTH.,#13328);
#13330=PRESENTATION_STYLE_ASSIGNMENT((#13329));
ENDSEC;
END-ISO-10303-21;
